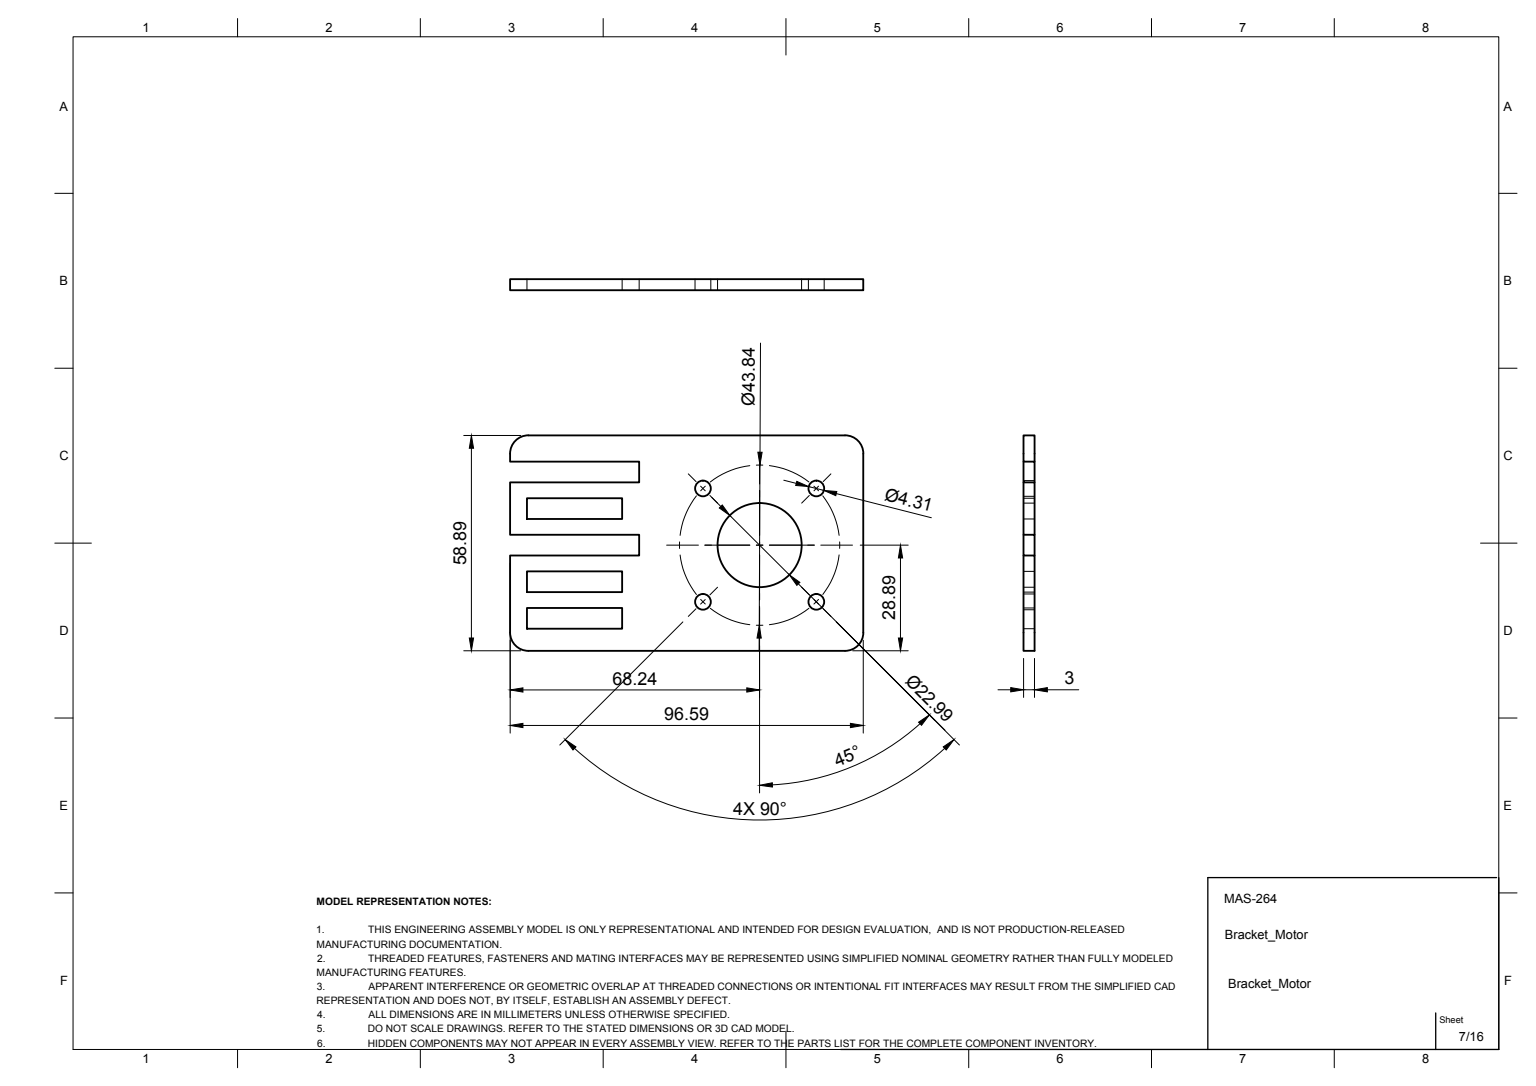
ISO-10303-21;
HEADER;
/* Generated by software containing ST-Developer
 * from STEP Tools, Inc. (www.steptools.com) 
 */

FILE_DESCRIPTION(
/* description */ (''),
/* implementation_level */ '2;1');

FILE_NAME(
/* name */ 'Bracket_Motor.step',
/* time_stamp */ '2026-10-12T15:37:13-07:00',
/* author */ (''),
/* organization */ (''),
/* preprocessor_version */ 'ST-DEVELOPER v20.2',
/* originating_system */ 'Autodesk Translation Framework v15.15.0.0',
/* authorisation */ '');

FILE_SCHEMA (('AUTOMOTIVE_DESIGN { 1 0 10303 214 3 1 1 }'));
ENDSEC;

DATA;
#10=MECHANICAL_DESIGN_GEOMETRIC_PRESENTATION_REPRESENTATION('',(#352),#36460);
#113=SHAPE_REPRESENTATION_RELATIONSHIP('SRR','None',#36525,#126);
#126=ADVANCED_BREP_SHAPE_REPRESENTATION('',(#384),#36454);
#182=FACE_BOUND('',#2191,.T.);
#183=FACE_BOUND('',#2192,.T.);
#184=FACE_BOUND('',#2193,.T.);
#185=FACE_BOUND('',#2194,.T.);
#186=FACE_BOUND('',#2195,.T.);
#187=FACE_BOUND('',#2196,.T.);
#188=FACE_BOUND('',#2197,.T.);
#189=FACE_BOUND('',#2198,.T.);
#190=FACE_BOUND('',#2200,.T.);
#191=FACE_BOUND('',#2201,.T.);
#192=FACE_BOUND('',#2202,.T.);
#193=FACE_BOUND('',#2203,.T.);
#194=FACE_BOUND('',#2204,.T.);
#195=FACE_BOUND('',#2205,.T.);
#196=FACE_BOUND('',#2206,.T.);
#197=FACE_BOUND('',#2207,.T.);
#352=STYLED_ITEM('',(#36596),#384);
#384=MANIFOLD_SOLID_BREP('Body1',#11288);
#634=PLANE('',#12139);
#635=PLANE('',#12140);
#636=PLANE('',#12141);
#637=PLANE('',#12142);
#638=PLANE('',#12143);
#639=PLANE('',#12144);
#640=PLANE('',#12145);
#641=PLANE('',#12146);
#642=PLANE('',#12153);
#643=PLANE('',#12154);
#644=PLANE('',#12155);
#645=PLANE('',#12156);
#646=PLANE('',#12163);
#647=PLANE('',#12164);
#648=PLANE('',#12165);
#649=PLANE('',#12166);
#650=PLANE('',#12167);
#651=PLANE('',#12168);
#652=PLANE('',#12169);
#653=PLANE('',#12170);
#654=PLANE('',#12171);
#655=PLANE('',#12175);
#656=PLANE('',#12179);
#657=PLANE('',#12183);
#658=PLANE('',#12187);
#659=PLANE('',#12188);
#1493=FACE_OUTER_BOUND('',#2157,.T.);
#1494=FACE_OUTER_BOUND('',#2158,.T.);
#1495=FACE_OUTER_BOUND('',#2159,.T.);
#1496=FACE_OUTER_BOUND('',#2160,.T.);
#1497=FACE_OUTER_BOUND('',#2161,.T.);
#1498=FACE_OUTER_BOUND('',#2162,.T.);
#1499=FACE_OUTER_BOUND('',#2163,.T.);
#1500=FACE_OUTER_BOUND('',#2164,.T.);
#1501=FACE_OUTER_BOUND('',#2165,.T.);
#1502=FACE_OUTER_BOUND('',#2166,.T.);
#1503=FACE_OUTER_BOUND('',#2167,.T.);
#1504=FACE_OUTER_BOUND('',#2168,.T.);
#1505=FACE_OUTER_BOUND('',#2169,.T.);
#1506=FACE_OUTER_BOUND('',#2170,.T.);
#1507=FACE_OUTER_BOUND('',#2171,.T.);
#1508=FACE_OUTER_BOUND('',#2172,.T.);
#1509=FACE_OUTER_BOUND('',#2173,.T.);
#1510=FACE_OUTER_BOUND('',#2174,.T.);
#1511=FACE_OUTER_BOUND('',#2175,.T.);
#1512=FACE_OUTER_BOUND('',#2176,.T.);
#1513=FACE_OUTER_BOUND('',#2177,.T.);
#1514=FACE_OUTER_BOUND('',#2178,.T.);
#1515=FACE_OUTER_BOUND('',#2179,.T.);
#1516=FACE_OUTER_BOUND('',#2180,.T.);
#1517=FACE_OUTER_BOUND('',#2181,.T.);
#1518=FACE_OUTER_BOUND('',#2182,.T.);
#1519=FACE_OUTER_BOUND('',#2183,.T.);
#1520=FACE_OUTER_BOUND('',#2184,.T.);
#1521=FACE_OUTER_BOUND('',#2185,.T.);
#1522=FACE_OUTER_BOUND('',#2186,.T.);
#1523=FACE_OUTER_BOUND('',#2187,.T.);
#1524=FACE_OUTER_BOUND('',#2188,.T.);
#1525=FACE_OUTER_BOUND('',#2189,.T.);
#1526=FACE_OUTER_BOUND('',#2190,.T.);
#1527=FACE_OUTER_BOUND('',#2199,.T.);
#2157=EDGE_LOOP('',(#9638,#9639,#9640,#9641));
#2158=EDGE_LOOP('',(#9642,#9643,#9644,#9645));
#2159=EDGE_LOOP('',(#9646,#9647,#9648,#9649));
#2160=EDGE_LOOP('',(#9650,#9651,#9652,#9653));
#2161=EDGE_LOOP('',(#9654,#9655,#9656,#9657));
#2162=EDGE_LOOP('',(#9658,#9659,#9660,#9661));
#2163=EDGE_LOOP('',(#9662,#9663,#9664,#9665));
#2164=EDGE_LOOP('',(#9666,#9667,#9668,#9669));
#2165=EDGE_LOOP('',(#9670,#9671,#9672,#9673));
#2166=EDGE_LOOP('',(#9674,#9675,#9676,#9677));
#2167=EDGE_LOOP('',(#9678,#9679,#9680,#9681));
#2168=EDGE_LOOP('',(#9682,#9683,#9684,#9685));
#2169=EDGE_LOOP('',(#9686,#9687,#9688,#9689));
#2170=EDGE_LOOP('',(#9690,#9691,#9692,#9693));
#2171=EDGE_LOOP('',(#9694,#9695,#9696,#9697));
#2172=EDGE_LOOP('',(#9698,#9699,#9700,#9701));
#2173=EDGE_LOOP('',(#9702,#9703,#9704,#9705));
#2174=EDGE_LOOP('',(#9706,#9707,#9708,#9709));
#2175=EDGE_LOOP('',(#9710,#9711,#9712,#9713));
#2176=EDGE_LOOP('',(#9714,#9715,#9716,#9717));
#2177=EDGE_LOOP('',(#9718,#9719,#9720,#9721));
#2178=EDGE_LOOP('',(#9722,#9723,#9724,#9725));
#2179=EDGE_LOOP('',(#9726,#9727,#9728,#9729));
#2180=EDGE_LOOP('',(#9730,#9731,#9732,#9733));
#2181=EDGE_LOOP('',(#9734,#9735,#9736,#9737));
#2182=EDGE_LOOP('',(#9738,#9739,#9740,#9741));
#2183=EDGE_LOOP('',(#9742,#9743,#9744,#9745));
#2184=EDGE_LOOP('',(#9746,#9747,#9748,#9749));
#2185=EDGE_LOOP('',(#9750,#9751,#9752,#9753));
#2186=EDGE_LOOP('',(#9754,#9755,#9756,#9757));
#2187=EDGE_LOOP('',(#9758,#9759,#9760,#9761));
#2188=EDGE_LOOP('',(#9762,#9763,#9764,#9765));
#2189=EDGE_LOOP('',(#9766,#9767,#9768,#9769));
#2190=EDGE_LOOP('',(#9770,#9771,#9772,#9773,#9774,#9775,#9776,#9777,#9778,
#9779,#9780,#9781,#9782,#9783,#9784,#9785));
#2191=EDGE_LOOP('',(#9786));
#2192=EDGE_LOOP('',(#9787));
#2193=EDGE_LOOP('',(#9788,#9789,#9790,#9791));
#2194=EDGE_LOOP('',(#9792));
#2195=EDGE_LOOP('',(#9793));
#2196=EDGE_LOOP('',(#9794,#9795,#9796,#9797));
#2197=EDGE_LOOP('',(#9798,#9799,#9800,#9801));
#2198=EDGE_LOOP('',(#9802));
#2199=EDGE_LOOP('',(#9803,#9804,#9805,#9806,#9807,#9808,#9809,#9810,#9811,
#9812,#9813,#9814,#9815,#9816,#9817,#9818));
#2200=EDGE_LOOP('',(#9819));
#2201=EDGE_LOOP('',(#9820));
#2202=EDGE_LOOP('',(#9821,#9822,#9823,#9824));
#2203=EDGE_LOOP('',(#9825));
#2204=EDGE_LOOP('',(#9826));
#2205=EDGE_LOOP('',(#9827,#9828,#9829,#9830));
#2206=EDGE_LOOP('',(#9831,#9832,#9833,#9834));
#2207=EDGE_LOOP('',(#9835));
#3086=LINE('',#35485,#4032);
#3087=LINE('',#35490,#4033);
#3088=LINE('',#35492,#4034);
#3089=LINE('',#35494,#4035);
#3090=LINE('',#35495,#4036);
#3091=LINE('',#35498,#4037);
#3092=LINE('',#35500,#4038);
#3093=LINE('',#35501,#4039);
#3094=LINE('',#35504,#4040);
#3095=LINE('',#35506,#4041);
#3096=LINE('',#35507,#4042);
#3097=LINE('',#35509,#4043);
#3098=LINE('',#35510,#4044);
#3099=LINE('',#35514,#4045);
#3100=LINE('',#35516,#4046);
#3101=LINE('',#35518,#4047);
#3102=LINE('',#35519,#4048);
#3103=LINE('',#35522,#4049);
#3104=LINE('',#35524,#4050);
#3105=LINE('',#35525,#4051);
#3106=LINE('',#35528,#4052);
#3107=LINE('',#35530,#4053);
#3108=LINE('',#35531,#4054);
#3109=LINE('',#35533,#4055);
#3110=LINE('',#35534,#4056);
#3111=LINE('',#35539,#4057);
#3112=LINE('',#35545,#4058);
#3113=LINE('',#35550,#4059);
#3114=LINE('',#35552,#4060);
#3115=LINE('',#35554,#4061);
#3116=LINE('',#35555,#4062);
#3117=LINE('',#35558,#4063);
#3118=LINE('',#35560,#4064);
#3119=LINE('',#35561,#4065);
#3120=LINE('',#35564,#4066);
#3121=LINE('',#35566,#4067);
#3122=LINE('',#35567,#4068);
#3123=LINE('',#35569,#4069);
#3124=LINE('',#35570,#4070);
#3125=LINE('',#35575,#4071);
#3126=LINE('',#35581,#4072);
#3127=LINE('',#35586,#4073);
#3128=LINE('',#35588,#4074);
#3129=LINE('',#35590,#4075);
#3130=LINE('',#35591,#4076);
#3131=LINE('',#35594,#4077);
#3132=LINE('',#35596,#4078);
#3133=LINE('',#35597,#4079);
#3134=LINE('',#35600,#4080);
#3135=LINE('',#35602,#4081);
#3136=LINE('',#35603,#4082);
#3137=LINE('',#35606,#4083);
#3138=LINE('',#35608,#4084);
#3139=LINE('',#35609,#4085);
#3140=LINE('',#35612,#4086);
#3141=LINE('',#35614,#4087);
#3142=LINE('',#35615,#4088);
#3143=LINE('',#35618,#4089);
#3144=LINE('',#35620,#4090);
#3145=LINE('',#35621,#4091);
#3146=LINE('',#35624,#4092);
#3147=LINE('',#35626,#4093);
#3148=LINE('',#35627,#4094);
#3149=LINE('',#35630,#4095);
#3150=LINE('',#35632,#4096);
#3151=LINE('',#35633,#4097);
#3152=LINE('',#35636,#4098);
#3153=LINE('',#35638,#4099);
#3154=LINE('',#35639,#4100);
#3155=LINE('',#35645,#4101);
#3156=LINE('',#35648,#4102);
#3157=LINE('',#35650,#4103);
#3158=LINE('',#35651,#4104);
#3159=LINE('',#35657,#4105);
#3160=LINE('',#35660,#4106);
#3161=LINE('',#35662,#4107);
#3162=LINE('',#35663,#4108);
#3163=LINE('',#35669,#4109);
#3164=LINE('',#35672,#4110);
#3165=LINE('',#35674,#4111);
#3166=LINE('',#35675,#4112);
#4032=VECTOR('',#14535,2.155);
#4033=VECTOR('',#14540,10.);
#4034=VECTOR('',#14541,10.);
#4035=VECTOR('',#14542,10.);
#4036=VECTOR('',#14543,10.);
#4037=VECTOR('',#14546,10.);
#4038=VECTOR('',#14547,10.);
#4039=VECTOR('',#14548,10.);
#4040=VECTOR('',#14551,10.);
#4041=VECTOR('',#14552,10.);
#4042=VECTOR('',#14553,10.);
#4043=VECTOR('',#14556,10.);
#4044=VECTOR('',#14557,10.);
#4045=VECTOR('',#14560,10.);
#4046=VECTOR('',#14561,10.);
#4047=VECTOR('',#14562,10.);
#4048=VECTOR('',#14563,10.);
#4049=VECTOR('',#14566,10.);
#4050=VECTOR('',#14567,10.);
#4051=VECTOR('',#14568,10.);
#4052=VECTOR('',#14571,10.);
#4053=VECTOR('',#14572,10.);
#4054=VECTOR('',#14573,10.);
#4055=VECTOR('',#14576,10.);
#4056=VECTOR('',#14577,10.);
#4057=VECTOR('',#14582,2.155);
#4058=VECTOR('',#14589,2.155);
#4059=VECTOR('',#14594,10.);
#4060=VECTOR('',#14595,10.);
#4061=VECTOR('',#14596,10.);
#4062=VECTOR('',#14597,10.);
#4063=VECTOR('',#14600,10.);
#4064=VECTOR('',#14601,10.);
#4065=VECTOR('',#14602,10.);
#4066=VECTOR('',#14605,10.);
#4067=VECTOR('',#14606,10.);
#4068=VECTOR('',#14607,10.);
#4069=VECTOR('',#14610,10.);
#4070=VECTOR('',#14611,10.);
#4071=VECTOR('',#14616,11.493);
#4072=VECTOR('',#14623,2.155);
#4073=VECTOR('',#14628,10.);
#4074=VECTOR('',#14629,10.);
#4075=VECTOR('',#14630,10.);
#4076=VECTOR('',#14631,10.);
#4077=VECTOR('',#14634,10.);
#4078=VECTOR('',#14635,10.);
#4079=VECTOR('',#14636,10.);
#4080=VECTOR('',#14639,10.);
#4081=VECTOR('',#14640,10.);
#4082=VECTOR('',#14641,10.);
#4083=VECTOR('',#14644,10.);
#4084=VECTOR('',#14645,10.);
#4085=VECTOR('',#14646,10.);
#4086=VECTOR('',#14649,10.);
#4087=VECTOR('',#14650,10.);
#4088=VECTOR('',#14651,10.);
#4089=VECTOR('',#14654,10.);
#4090=VECTOR('',#14655,10.);
#4091=VECTOR('',#14656,10.);
#4092=VECTOR('',#14659,10.);
#4093=VECTOR('',#14660,10.);
#4094=VECTOR('',#14661,10.);
#4095=VECTOR('',#14664,10.);
#4096=VECTOR('',#14665,10.);
#4097=VECTOR('',#14666,10.);
#4098=VECTOR('',#14669,10.);
#4099=VECTOR('',#14670,10.);
#4100=VECTOR('',#14671,10.);
#4101=VECTOR('',#14678,10.);
#4102=VECTOR('',#14681,10.);
#4103=VECTOR('',#14682,10.);
#4104=VECTOR('',#14683,10.);
#4105=VECTOR('',#14690,10.);
#4106=VECTOR('',#14693,10.);
#4107=VECTOR('',#14694,10.);
#4108=VECTOR('',#14695,10.);
#4109=VECTOR('',#14702,10.);
#4110=VECTOR('',#14705,10.);
#4111=VECTOR('',#14706,10.);
#4112=VECTOR('',#14707,10.);
#4461=CIRCLE('',#12137,2.155);
#4462=CIRCLE('',#12138,2.155);
#4463=CIRCLE('',#12148,2.155);
#4464=CIRCLE('',#12149,2.155);
#4465=CIRCLE('',#12151,2.155);
#4466=CIRCLE('',#12152,2.155);
#4467=CIRCLE('',#12158,11.493);
#4468=CIRCLE('',#12159,11.493);
#4469=CIRCLE('',#12161,2.155);
#4470=CIRCLE('',#12162,2.155);
#4471=CIRCLE('',#12173,5.);
#4472=CIRCLE('',#12174,5.);
#4473=CIRCLE('',#12177,5.00000000000002);
#4474=CIRCLE('',#12178,5.00000000000002);
#4475=CIRCLE('',#12181,5.);
#4476=CIRCLE('',#12182,5.);
#4477=CIRCLE('',#12185,4.99999999999999);
#4478=CIRCLE('',#12186,4.99999999999999);
#5395=VERTEX_POINT('',#35482);
#5396=VERTEX_POINT('',#35484);
#5397=VERTEX_POINT('',#35488);
#5398=VERTEX_POINT('',#35489);
#5399=VERTEX_POINT('',#35491);
#5400=VERTEX_POINT('',#35493);
#5401=VERTEX_POINT('',#35497);
#5402=VERTEX_POINT('',#35499);
#5403=VERTEX_POINT('',#35503);
#5404=VERTEX_POINT('',#35505);
#5405=VERTEX_POINT('',#35512);
#5406=VERTEX_POINT('',#35513);
#5407=VERTEX_POINT('',#35515);
#5408=VERTEX_POINT('',#35517);
#5409=VERTEX_POINT('',#35521);
#5410=VERTEX_POINT('',#35523);
#5411=VERTEX_POINT('',#35527);
#5412=VERTEX_POINT('',#35529);
#5413=VERTEX_POINT('',#35536);
#5414=VERTEX_POINT('',#35538);
#5415=VERTEX_POINT('',#35542);
#5416=VERTEX_POINT('',#35544);
#5417=VERTEX_POINT('',#35548);
#5418=VERTEX_POINT('',#35549);
#5419=VERTEX_POINT('',#35551);
#5420=VERTEX_POINT('',#35553);
#5421=VERTEX_POINT('',#35557);
#5422=VERTEX_POINT('',#35559);
#5423=VERTEX_POINT('',#35563);
#5424=VERTEX_POINT('',#35565);
#5425=VERTEX_POINT('',#35572);
#5426=VERTEX_POINT('',#35574);
#5427=VERTEX_POINT('',#35578);
#5428=VERTEX_POINT('',#35580);
#5429=VERTEX_POINT('',#35584);
#5430=VERTEX_POINT('',#35585);
#5431=VERTEX_POINT('',#35587);
#5432=VERTEX_POINT('',#35589);
#5433=VERTEX_POINT('',#35593);
#5434=VERTEX_POINT('',#35595);
#5435=VERTEX_POINT('',#35599);
#5436=VERTEX_POINT('',#35601);
#5437=VERTEX_POINT('',#35605);
#5438=VERTEX_POINT('',#35607);
#5439=VERTEX_POINT('',#35611);
#5440=VERTEX_POINT('',#35613);
#5441=VERTEX_POINT('',#35617);
#5442=VERTEX_POINT('',#35619);
#5443=VERTEX_POINT('',#35623);
#5444=VERTEX_POINT('',#35625);
#5445=VERTEX_POINT('',#35629);
#5446=VERTEX_POINT('',#35631);
#5447=VERTEX_POINT('',#35635);
#5448=VERTEX_POINT('',#35637);
#5449=VERTEX_POINT('',#35641);
#5450=VERTEX_POINT('',#35643);
#5451=VERTEX_POINT('',#35647);
#5452=VERTEX_POINT('',#35649);
#5453=VERTEX_POINT('',#35653);
#5454=VERTEX_POINT('',#35655);
#5455=VERTEX_POINT('',#35659);
#5456=VERTEX_POINT('',#35661);
#5457=VERTEX_POINT('',#35665);
#5458=VERTEX_POINT('',#35667);
#5459=VERTEX_POINT('',#35671);
#5460=VERTEX_POINT('',#35673);
#6850=EDGE_CURVE('',#5395,#5395,#4461,.T.);
#6851=EDGE_CURVE('',#5395,#5396,#3086,.T.);
#6852=EDGE_CURVE('',#5396,#5396,#4462,.T.);
#6853=EDGE_CURVE('',#5397,#5398,#3087,.T.);
#6854=EDGE_CURVE('',#5398,#5399,#3088,.T.);
#6855=EDGE_CURVE('',#5400,#5399,#3089,.T.);
#6856=EDGE_CURVE('',#5397,#5400,#3090,.T.);
#6857=EDGE_CURVE('',#5401,#5397,#3091,.T.);
#6858=EDGE_CURVE('',#5402,#5400,#3092,.T.);
#6859=EDGE_CURVE('',#5401,#5402,#3093,.T.);
#6860=EDGE_CURVE('',#5403,#5401,#3094,.T.);
#6861=EDGE_CURVE('',#5404,#5402,#3095,.T.);
#6862=EDGE_CURVE('',#5403,#5404,#3096,.T.);
#6863=EDGE_CURVE('',#5398,#5403,#3097,.T.);
#6864=EDGE_CURVE('',#5399,#5404,#3098,.T.);
#6865=EDGE_CURVE('',#5405,#5406,#3099,.T.);
#6866=EDGE_CURVE('',#5406,#5407,#3100,.T.);
#6867=EDGE_CURVE('',#5408,#5407,#3101,.T.);
#6868=EDGE_CURVE('',#5405,#5408,#3102,.T.);
#6869=EDGE_CURVE('',#5409,#5405,#3103,.T.);
#6870=EDGE_CURVE('',#5410,#5408,#3104,.T.);
#6871=EDGE_CURVE('',#5409,#5410,#3105,.T.);
#6872=EDGE_CURVE('',#5411,#5409,#3106,.T.);
#6873=EDGE_CURVE('',#5412,#5410,#3107,.T.);
#6874=EDGE_CURVE('',#5411,#5412,#3108,.T.);
#6875=EDGE_CURVE('',#5406,#5411,#3109,.T.);
#6876=EDGE_CURVE('',#5407,#5412,#3110,.T.);
#6877=EDGE_CURVE('',#5413,#5413,#4463,.T.);
#6878=EDGE_CURVE('',#5413,#5414,#3111,.T.);
#6879=EDGE_CURVE('',#5414,#5414,#4464,.T.);
#6880=EDGE_CURVE('',#5415,#5415,#4465,.T.);
#6881=EDGE_CURVE('',#5415,#5416,#3112,.T.);
#6882=EDGE_CURVE('',#5416,#5416,#4466,.T.);
#6883=EDGE_CURVE('',#5417,#5418,#3113,.T.);
#6884=EDGE_CURVE('',#5418,#5419,#3114,.T.);
#6885=EDGE_CURVE('',#5420,#5419,#3115,.T.);
#6886=EDGE_CURVE('',#5417,#5420,#3116,.T.);
#6887=EDGE_CURVE('',#5421,#5417,#3117,.T.);
#6888=EDGE_CURVE('',#5422,#5420,#3118,.T.);
#6889=EDGE_CURVE('',#5421,#5422,#3119,.T.);
#6890=EDGE_CURVE('',#5423,#5421,#3120,.T.);
#6891=EDGE_CURVE('',#5424,#5422,#3121,.T.);
#6892=EDGE_CURVE('',#5423,#5424,#3122,.T.);
#6893=EDGE_CURVE('',#5418,#5423,#3123,.T.);
#6894=EDGE_CURVE('',#5419,#5424,#3124,.T.);
#6895=EDGE_CURVE('',#5425,#5425,#4467,.T.);
#6896=EDGE_CURVE('',#5425,#5426,#3125,.T.);
#6897=EDGE_CURVE('',#5426,#5426,#4468,.T.);
#6898=EDGE_CURVE('',#5427,#5427,#4469,.T.);
#6899=EDGE_CURVE('',#5427,#5428,#3126,.T.);
#6900=EDGE_CURVE('',#5428,#5428,#4470,.T.);
#6901=EDGE_CURVE('',#5429,#5430,#3127,.T.);
#6902=EDGE_CURVE('',#5429,#5431,#3128,.T.);
#6903=EDGE_CURVE('',#5432,#5431,#3129,.T.);
#6904=EDGE_CURVE('',#5430,#5432,#3130,.T.);
#6905=EDGE_CURVE('',#5430,#5433,#3131,.T.);
#6906=EDGE_CURVE('',#5434,#5432,#3132,.T.);
#6907=EDGE_CURVE('',#5433,#5434,#3133,.T.);
#6908=EDGE_CURVE('',#5433,#5435,#3134,.T.);
#6909=EDGE_CURVE('',#5436,#5434,#3135,.T.);
#6910=EDGE_CURVE('',#5435,#5436,#3136,.T.);
#6911=EDGE_CURVE('',#5435,#5437,#3137,.T.);
#6912=EDGE_CURVE('',#5438,#5436,#3138,.T.);
#6913=EDGE_CURVE('',#5437,#5438,#3139,.T.);
#6914=EDGE_CURVE('',#5437,#5439,#3140,.T.);
#6915=EDGE_CURVE('',#5440,#5438,#3141,.T.);
#6916=EDGE_CURVE('',#5439,#5440,#3142,.T.);
#6917=EDGE_CURVE('',#5439,#5441,#3143,.T.);
#6918=EDGE_CURVE('',#5442,#5440,#3144,.T.);
#6919=EDGE_CURVE('',#5441,#5442,#3145,.T.);
#6920=EDGE_CURVE('',#5441,#5443,#3146,.T.);
#6921=EDGE_CURVE('',#5444,#5442,#3147,.T.);
#6922=EDGE_CURVE('',#5443,#5444,#3148,.T.);
#6923=EDGE_CURVE('',#5443,#5445,#3149,.T.);
#6924=EDGE_CURVE('',#5446,#5444,#3150,.T.);
#6925=EDGE_CURVE('',#5445,#5446,#3151,.T.);
#6926=EDGE_CURVE('',#5445,#5447,#3152,.T.);
#6927=EDGE_CURVE('',#5448,#5446,#3153,.T.);
#6928=EDGE_CURVE('',#5447,#5448,#3154,.T.);
#6929=EDGE_CURVE('',#5449,#5447,#4471,.T.);
#6930=EDGE_CURVE('',#5450,#5448,#4472,.T.);
#6931=EDGE_CURVE('',#5449,#5450,#3155,.T.);
#6932=EDGE_CURVE('',#5449,#5451,#3156,.T.);
#6933=EDGE_CURVE('',#5452,#5450,#3157,.T.);
#6934=EDGE_CURVE('',#5451,#5452,#3158,.T.);
#6935=EDGE_CURVE('',#5453,#5451,#4473,.T.);
#6936=EDGE_CURVE('',#5454,#5452,#4474,.T.);
#6937=EDGE_CURVE('',#5453,#5454,#3159,.T.);
#6938=EDGE_CURVE('',#5453,#5455,#3160,.T.);
#6939=EDGE_CURVE('',#5456,#5454,#3161,.T.);
#6940=EDGE_CURVE('',#5455,#5456,#3162,.T.);
#6941=EDGE_CURVE('',#5457,#5455,#4475,.T.);
#6942=EDGE_CURVE('',#5458,#5456,#4476,.T.);
#6943=EDGE_CURVE('',#5457,#5458,#3163,.T.);
#6944=EDGE_CURVE('',#5457,#5459,#3164,.T.);
#6945=EDGE_CURVE('',#5460,#5458,#3165,.T.);
#6946=EDGE_CURVE('',#5459,#5460,#3166,.T.);
#6947=EDGE_CURVE('',#5429,#5459,#4477,.T.);
#6948=EDGE_CURVE('',#5431,#5460,#4478,.T.);
#9638=ORIENTED_EDGE('',*,*,#6850,.T.);
#9639=ORIENTED_EDGE('',*,*,#6851,.T.);
#9640=ORIENTED_EDGE('',*,*,#6852,.F.);
#9641=ORIENTED_EDGE('',*,*,#6851,.F.);
#9642=ORIENTED_EDGE('',*,*,#6853,.T.);
#9643=ORIENTED_EDGE('',*,*,#6854,.T.);
#9644=ORIENTED_EDGE('',*,*,#6855,.F.);
#9645=ORIENTED_EDGE('',*,*,#6856,.F.);
#9646=ORIENTED_EDGE('',*,*,#6857,.T.);
#9647=ORIENTED_EDGE('',*,*,#6856,.T.);
#9648=ORIENTED_EDGE('',*,*,#6858,.F.);
#9649=ORIENTED_EDGE('',*,*,#6859,.F.);
#9650=ORIENTED_EDGE('',*,*,#6860,.T.);
#9651=ORIENTED_EDGE('',*,*,#6859,.T.);
#9652=ORIENTED_EDGE('',*,*,#6861,.F.);
#9653=ORIENTED_EDGE('',*,*,#6862,.F.);
#9654=ORIENTED_EDGE('',*,*,#6863,.T.);
#9655=ORIENTED_EDGE('',*,*,#6862,.T.);
#9656=ORIENTED_EDGE('',*,*,#6864,.F.);
#9657=ORIENTED_EDGE('',*,*,#6854,.F.);
#9658=ORIENTED_EDGE('',*,*,#6865,.T.);
#9659=ORIENTED_EDGE('',*,*,#6866,.T.);
#9660=ORIENTED_EDGE('',*,*,#6867,.F.);
#9661=ORIENTED_EDGE('',*,*,#6868,.F.);
#9662=ORIENTED_EDGE('',*,*,#6869,.T.);
#9663=ORIENTED_EDGE('',*,*,#6868,.T.);
#9664=ORIENTED_EDGE('',*,*,#6870,.F.);
#9665=ORIENTED_EDGE('',*,*,#6871,.F.);
#9666=ORIENTED_EDGE('',*,*,#6872,.T.);
#9667=ORIENTED_EDGE('',*,*,#6871,.T.);
#9668=ORIENTED_EDGE('',*,*,#6873,.F.);
#9669=ORIENTED_EDGE('',*,*,#6874,.F.);
#9670=ORIENTED_EDGE('',*,*,#6875,.T.);
#9671=ORIENTED_EDGE('',*,*,#6874,.T.);
#9672=ORIENTED_EDGE('',*,*,#6876,.F.);
#9673=ORIENTED_EDGE('',*,*,#6866,.F.);
#9674=ORIENTED_EDGE('',*,*,#6877,.T.);
#9675=ORIENTED_EDGE('',*,*,#6878,.T.);
#9676=ORIENTED_EDGE('',*,*,#6879,.F.);
#9677=ORIENTED_EDGE('',*,*,#6878,.F.);
#9678=ORIENTED_EDGE('',*,*,#6880,.T.);
#9679=ORIENTED_EDGE('',*,*,#6881,.T.);
#9680=ORIENTED_EDGE('',*,*,#6882,.F.);
#9681=ORIENTED_EDGE('',*,*,#6881,.F.);
#9682=ORIENTED_EDGE('',*,*,#6883,.T.);
#9683=ORIENTED_EDGE('',*,*,#6884,.T.);
#9684=ORIENTED_EDGE('',*,*,#6885,.F.);
#9685=ORIENTED_EDGE('',*,*,#6886,.F.);
#9686=ORIENTED_EDGE('',*,*,#6887,.T.);
#9687=ORIENTED_EDGE('',*,*,#6886,.T.);
#9688=ORIENTED_EDGE('',*,*,#6888,.F.);
#9689=ORIENTED_EDGE('',*,*,#6889,.F.);
#9690=ORIENTED_EDGE('',*,*,#6890,.T.);
#9691=ORIENTED_EDGE('',*,*,#6889,.T.);
#9692=ORIENTED_EDGE('',*,*,#6891,.F.);
#9693=ORIENTED_EDGE('',*,*,#6892,.F.);
#9694=ORIENTED_EDGE('',*,*,#6893,.T.);
#9695=ORIENTED_EDGE('',*,*,#6892,.T.);
#9696=ORIENTED_EDGE('',*,*,#6894,.F.);
#9697=ORIENTED_EDGE('',*,*,#6884,.F.);
#9698=ORIENTED_EDGE('',*,*,#6895,.T.);
#9699=ORIENTED_EDGE('',*,*,#6896,.T.);
#9700=ORIENTED_EDGE('',*,*,#6897,.F.);
#9701=ORIENTED_EDGE('',*,*,#6896,.F.);
#9702=ORIENTED_EDGE('',*,*,#6898,.T.);
#9703=ORIENTED_EDGE('',*,*,#6899,.T.);
#9704=ORIENTED_EDGE('',*,*,#6900,.F.);
#9705=ORIENTED_EDGE('',*,*,#6899,.F.);
#9706=ORIENTED_EDGE('',*,*,#6901,.F.);
#9707=ORIENTED_EDGE('',*,*,#6902,.T.);
#9708=ORIENTED_EDGE('',*,*,#6903,.F.);
#9709=ORIENTED_EDGE('',*,*,#6904,.F.);
#9710=ORIENTED_EDGE('',*,*,#6905,.F.);
#9711=ORIENTED_EDGE('',*,*,#6904,.T.);
#9712=ORIENTED_EDGE('',*,*,#6906,.F.);
#9713=ORIENTED_EDGE('',*,*,#6907,.F.);
#9714=ORIENTED_EDGE('',*,*,#6908,.F.);
#9715=ORIENTED_EDGE('',*,*,#6907,.T.);
#9716=ORIENTED_EDGE('',*,*,#6909,.F.);
#9717=ORIENTED_EDGE('',*,*,#6910,.F.);
#9718=ORIENTED_EDGE('',*,*,#6911,.F.);
#9719=ORIENTED_EDGE('',*,*,#6910,.T.);
#9720=ORIENTED_EDGE('',*,*,#6912,.F.);
#9721=ORIENTED_EDGE('',*,*,#6913,.F.);
#9722=ORIENTED_EDGE('',*,*,#6914,.F.);
#9723=ORIENTED_EDGE('',*,*,#6913,.T.);
#9724=ORIENTED_EDGE('',*,*,#6915,.F.);
#9725=ORIENTED_EDGE('',*,*,#6916,.F.);
#9726=ORIENTED_EDGE('',*,*,#6917,.F.);
#9727=ORIENTED_EDGE('',*,*,#6916,.T.);
#9728=ORIENTED_EDGE('',*,*,#6918,.F.);
#9729=ORIENTED_EDGE('',*,*,#6919,.F.);
#9730=ORIENTED_EDGE('',*,*,#6920,.F.);
#9731=ORIENTED_EDGE('',*,*,#6919,.T.);
#9732=ORIENTED_EDGE('',*,*,#6921,.F.);
#9733=ORIENTED_EDGE('',*,*,#6922,.F.);
#9734=ORIENTED_EDGE('',*,*,#6923,.F.);
#9735=ORIENTED_EDGE('',*,*,#6922,.T.);
#9736=ORIENTED_EDGE('',*,*,#6924,.F.);
#9737=ORIENTED_EDGE('',*,*,#6925,.F.);
#9738=ORIENTED_EDGE('',*,*,#6926,.F.);
#9739=ORIENTED_EDGE('',*,*,#6925,.T.);
#9740=ORIENTED_EDGE('',*,*,#6927,.F.);
#9741=ORIENTED_EDGE('',*,*,#6928,.F.);
#9742=ORIENTED_EDGE('',*,*,#6929,.T.);
#9743=ORIENTED_EDGE('',*,*,#6928,.T.);
#9744=ORIENTED_EDGE('',*,*,#6930,.F.);
#9745=ORIENTED_EDGE('',*,*,#6931,.F.);
#9746=ORIENTED_EDGE('',*,*,#6932,.F.);
#9747=ORIENTED_EDGE('',*,*,#6931,.T.);
#9748=ORIENTED_EDGE('',*,*,#6933,.F.);
#9749=ORIENTED_EDGE('',*,*,#6934,.F.);
#9750=ORIENTED_EDGE('',*,*,#6935,.T.);
#9751=ORIENTED_EDGE('',*,*,#6934,.T.);
#9752=ORIENTED_EDGE('',*,*,#6936,.F.);
#9753=ORIENTED_EDGE('',*,*,#6937,.F.);
#9754=ORIENTED_EDGE('',*,*,#6938,.F.);
#9755=ORIENTED_EDGE('',*,*,#6937,.T.);
#9756=ORIENTED_EDGE('',*,*,#6939,.F.);
#9757=ORIENTED_EDGE('',*,*,#6940,.F.);
#9758=ORIENTED_EDGE('',*,*,#6941,.T.);
#9759=ORIENTED_EDGE('',*,*,#6940,.T.);
#9760=ORIENTED_EDGE('',*,*,#6942,.F.);
#9761=ORIENTED_EDGE('',*,*,#6943,.F.);
#9762=ORIENTED_EDGE('',*,*,#6944,.F.);
#9763=ORIENTED_EDGE('',*,*,#6943,.T.);
#9764=ORIENTED_EDGE('',*,*,#6945,.F.);
#9765=ORIENTED_EDGE('',*,*,#6946,.F.);
#9766=ORIENTED_EDGE('',*,*,#6947,.T.);
#9767=ORIENTED_EDGE('',*,*,#6946,.T.);
#9768=ORIENTED_EDGE('',*,*,#6948,.F.);
#9769=ORIENTED_EDGE('',*,*,#6902,.F.);
#9770=ORIENTED_EDGE('',*,*,#6948,.T.);
#9771=ORIENTED_EDGE('',*,*,#6945,.T.);
#9772=ORIENTED_EDGE('',*,*,#6942,.T.);
#9773=ORIENTED_EDGE('',*,*,#6939,.T.);
#9774=ORIENTED_EDGE('',*,*,#6936,.T.);
#9775=ORIENTED_EDGE('',*,*,#6933,.T.);
#9776=ORIENTED_EDGE('',*,*,#6930,.T.);
#9777=ORIENTED_EDGE('',*,*,#6927,.T.);
#9778=ORIENTED_EDGE('',*,*,#6924,.T.);
#9779=ORIENTED_EDGE('',*,*,#6921,.T.);
#9780=ORIENTED_EDGE('',*,*,#6918,.T.);
#9781=ORIENTED_EDGE('',*,*,#6915,.T.);
#9782=ORIENTED_EDGE('',*,*,#6912,.T.);
#9783=ORIENTED_EDGE('',*,*,#6909,.T.);
#9784=ORIENTED_EDGE('',*,*,#6906,.T.);
#9785=ORIENTED_EDGE('',*,*,#6903,.T.);
#9786=ORIENTED_EDGE('',*,*,#6900,.T.);
#9787=ORIENTED_EDGE('',*,*,#6897,.T.);
#9788=ORIENTED_EDGE('',*,*,#6894,.T.);
#9789=ORIENTED_EDGE('',*,*,#6891,.T.);
#9790=ORIENTED_EDGE('',*,*,#6888,.T.);
#9791=ORIENTED_EDGE('',*,*,#6885,.T.);
#9792=ORIENTED_EDGE('',*,*,#6882,.T.);
#9793=ORIENTED_EDGE('',*,*,#6879,.T.);
#9794=ORIENTED_EDGE('',*,*,#6876,.T.);
#9795=ORIENTED_EDGE('',*,*,#6873,.T.);
#9796=ORIENTED_EDGE('',*,*,#6870,.T.);
#9797=ORIENTED_EDGE('',*,*,#6867,.T.);
#9798=ORIENTED_EDGE('',*,*,#6864,.T.);
#9799=ORIENTED_EDGE('',*,*,#6861,.T.);
#9800=ORIENTED_EDGE('',*,*,#6858,.T.);
#9801=ORIENTED_EDGE('',*,*,#6855,.T.);
#9802=ORIENTED_EDGE('',*,*,#6852,.T.);
#9803=ORIENTED_EDGE('',*,*,#6947,.F.);
#9804=ORIENTED_EDGE('',*,*,#6901,.T.);
#9805=ORIENTED_EDGE('',*,*,#6905,.T.);
#9806=ORIENTED_EDGE('',*,*,#6908,.T.);
#9807=ORIENTED_EDGE('',*,*,#6911,.T.);
#9808=ORIENTED_EDGE('',*,*,#6914,.T.);
#9809=ORIENTED_EDGE('',*,*,#6917,.T.);
#9810=ORIENTED_EDGE('',*,*,#6920,.T.);
#9811=ORIENTED_EDGE('',*,*,#6923,.T.);
#9812=ORIENTED_EDGE('',*,*,#6926,.T.);
#9813=ORIENTED_EDGE('',*,*,#6929,.F.);
#9814=ORIENTED_EDGE('',*,*,#6932,.T.);
#9815=ORIENTED_EDGE('',*,*,#6935,.F.);
#9816=ORIENTED_EDGE('',*,*,#6938,.T.);
#9817=ORIENTED_EDGE('',*,*,#6941,.F.);
#9818=ORIENTED_EDGE('',*,*,#6944,.T.);
#9819=ORIENTED_EDGE('',*,*,#6898,.F.);
#9820=ORIENTED_EDGE('',*,*,#6895,.F.);
#9821=ORIENTED_EDGE('',*,*,#6893,.F.);
#9822=ORIENTED_EDGE('',*,*,#6883,.F.);
#9823=ORIENTED_EDGE('',*,*,#6887,.F.);
#9824=ORIENTED_EDGE('',*,*,#6890,.F.);
#9825=ORIENTED_EDGE('',*,*,#6880,.F.);
#9826=ORIENTED_EDGE('',*,*,#6877,.F.);
#9827=ORIENTED_EDGE('',*,*,#6875,.F.);
#9828=ORIENTED_EDGE('',*,*,#6865,.F.);
#9829=ORIENTED_EDGE('',*,*,#6869,.F.);
#9830=ORIENTED_EDGE('',*,*,#6872,.F.);
#9831=ORIENTED_EDGE('',*,*,#6863,.F.);
#9832=ORIENTED_EDGE('',*,*,#6853,.F.);
#9833=ORIENTED_EDGE('',*,*,#6857,.F.);
#9834=ORIENTED_EDGE('',*,*,#6860,.F.);
#9835=ORIENTED_EDGE('',*,*,#6850,.F.);
#10583=CYLINDRICAL_SURFACE('',#12136,2.155);
#10584=CYLINDRICAL_SURFACE('',#12147,2.155);
#10585=CYLINDRICAL_SURFACE('',#12150,2.155);
#10586=CYLINDRICAL_SURFACE('',#12157,11.493);
#10587=CYLINDRICAL_SURFACE('',#12160,2.155);
#10588=CYLINDRICAL_SURFACE('',#12172,5.);
#10589=CYLINDRICAL_SURFACE('',#12176,5.00000000000002);
#10590=CYLINDRICAL_SURFACE('',#12180,5.);
#10591=CYLINDRICAL_SURFACE('',#12184,4.99999999999999);
#11114=ADVANCED_FACE('',(#1493),#10583,.F.);
#11115=ADVANCED_FACE('',(#1494),#634,.T.);
#11116=ADVANCED_FACE('',(#1495),#635,.T.);
#11117=ADVANCED_FACE('',(#1496),#636,.T.);
#11118=ADVANCED_FACE('',(#1497),#637,.T.);
#11119=ADVANCED_FACE('',(#1498),#638,.T.);
#11120=ADVANCED_FACE('',(#1499),#639,.T.);
#11121=ADVANCED_FACE('',(#1500),#640,.T.);
#11122=ADVANCED_FACE('',(#1501),#641,.T.);
#11123=ADVANCED_FACE('',(#1502),#10584,.F.);
#11124=ADVANCED_FACE('',(#1503),#10585,.F.);
#11125=ADVANCED_FACE('',(#1504),#642,.T.);
#11126=ADVANCED_FACE('',(#1505),#643,.T.);
#11127=ADVANCED_FACE('',(#1506),#644,.T.);
#11128=ADVANCED_FACE('',(#1507),#645,.T.);
#11129=ADVANCED_FACE('',(#1508),#10586,.F.);
#11130=ADVANCED_FACE('',(#1509),#10587,.F.);
#11131=ADVANCED_FACE('',(#1510),#646,.T.);
#11132=ADVANCED_FACE('',(#1511),#647,.T.);
#11133=ADVANCED_FACE('',(#1512),#648,.T.);
#11134=ADVANCED_FACE('',(#1513),#649,.T.);
#11135=ADVANCED_FACE('',(#1514),#650,.T.);
#11136=ADVANCED_FACE('',(#1515),#651,.T.);
#11137=ADVANCED_FACE('',(#1516),#652,.T.);
#11138=ADVANCED_FACE('',(#1517),#653,.T.);
#11139=ADVANCED_FACE('',(#1518),#654,.T.);
#11140=ADVANCED_FACE('',(#1519),#10588,.T.);
#11141=ADVANCED_FACE('',(#1520),#655,.T.);
#11142=ADVANCED_FACE('',(#1521),#10589,.T.);
#11143=ADVANCED_FACE('',(#1522),#656,.T.);
#11144=ADVANCED_FACE('',(#1523),#10590,.T.);
#11145=ADVANCED_FACE('',(#1524),#657,.T.);
#11146=ADVANCED_FACE('',(#1525),#10591,.T.);
#11147=ADVANCED_FACE('',(#1526,#182,#183,#184,#185,#186,#187,#188,#189),
#658,.T.);
#11148=ADVANCED_FACE('',(#1527,#190,#191,#192,#193,#194,#195,#196,#197),
#659,.F.);
#11288=CLOSED_SHELL('',(#11114,#11115,#11116,#11117,#11118,#11119,#11120,
#11121,#11122,#11123,#11124,#11125,#11126,#11127,#11128,#11129,#11130,#11131,
#11132,#11133,#11134,#11135,#11136,#11137,#11138,#11139,#11140,#11141,#11142,
#11143,#11144,#11145,#11146,#11147,#11148));
#12135=AXIS2_PLACEMENT_3D('',#35480,#14529,#14530);
#12136=AXIS2_PLACEMENT_3D('',#35481,#14531,#14532);
#12137=AXIS2_PLACEMENT_3D('',#35483,#14533,#14534);
#12138=AXIS2_PLACEMENT_3D('',#35486,#14536,#14537);
#12139=AXIS2_PLACEMENT_3D('',#35487,#14538,#14539);
#12140=AXIS2_PLACEMENT_3D('',#35496,#14544,#14545);
#12141=AXIS2_PLACEMENT_3D('',#35502,#14549,#14550);
#12142=AXIS2_PLACEMENT_3D('',#35508,#14554,#14555);
#12143=AXIS2_PLACEMENT_3D('',#35511,#14558,#14559);
#12144=AXIS2_PLACEMENT_3D('',#35520,#14564,#14565);
#12145=AXIS2_PLACEMENT_3D('',#35526,#14569,#14570);
#12146=AXIS2_PLACEMENT_3D('',#35532,#14574,#14575);
#12147=AXIS2_PLACEMENT_3D('',#35535,#14578,#14579);
#12148=AXIS2_PLACEMENT_3D('',#35537,#14580,#14581);
#12149=AXIS2_PLACEMENT_3D('',#35540,#14583,#14584);
#12150=AXIS2_PLACEMENT_3D('',#35541,#14585,#14586);
#12151=AXIS2_PLACEMENT_3D('',#35543,#14587,#14588);
#12152=AXIS2_PLACEMENT_3D('',#35546,#14590,#14591);
#12153=AXIS2_PLACEMENT_3D('',#35547,#14592,#14593);
#12154=AXIS2_PLACEMENT_3D('',#35556,#14598,#14599);
#12155=AXIS2_PLACEMENT_3D('',#35562,#14603,#14604);
#12156=AXIS2_PLACEMENT_3D('',#35568,#14608,#14609);
#12157=AXIS2_PLACEMENT_3D('',#35571,#14612,#14613);
#12158=AXIS2_PLACEMENT_3D('',#35573,#14614,#14615);
#12159=AXIS2_PLACEMENT_3D('',#35576,#14617,#14618);
#12160=AXIS2_PLACEMENT_3D('',#35577,#14619,#14620);
#12161=AXIS2_PLACEMENT_3D('',#35579,#14621,#14622);
#12162=AXIS2_PLACEMENT_3D('',#35582,#14624,#14625);
#12163=AXIS2_PLACEMENT_3D('',#35583,#14626,#14627);
#12164=AXIS2_PLACEMENT_3D('',#35592,#14632,#14633);
#12165=AXIS2_PLACEMENT_3D('',#35598,#14637,#14638);
#12166=AXIS2_PLACEMENT_3D('',#35604,#14642,#14643);
#12167=AXIS2_PLACEMENT_3D('',#35610,#14647,#14648);
#12168=AXIS2_PLACEMENT_3D('',#35616,#14652,#14653);
#12169=AXIS2_PLACEMENT_3D('',#35622,#14657,#14658);
#12170=AXIS2_PLACEMENT_3D('',#35628,#14662,#14663);
#12171=AXIS2_PLACEMENT_3D('',#35634,#14667,#14668);
#12172=AXIS2_PLACEMENT_3D('',#35640,#14672,#14673);
#12173=AXIS2_PLACEMENT_3D('',#35642,#14674,#14675);
#12174=AXIS2_PLACEMENT_3D('',#35644,#14676,#14677);
#12175=AXIS2_PLACEMENT_3D('',#35646,#14679,#14680);
#12176=AXIS2_PLACEMENT_3D('',#35652,#14684,#14685);
#12177=AXIS2_PLACEMENT_3D('',#35654,#14686,#14687);
#12178=AXIS2_PLACEMENT_3D('',#35656,#14688,#14689);
#12179=AXIS2_PLACEMENT_3D('',#35658,#14691,#14692);
#12180=AXIS2_PLACEMENT_3D('',#35664,#14696,#14697);
#12181=AXIS2_PLACEMENT_3D('',#35666,#14698,#14699);
#12182=AXIS2_PLACEMENT_3D('',#35668,#14700,#14701);
#12183=AXIS2_PLACEMENT_3D('',#35670,#14703,#14704);
#12184=AXIS2_PLACEMENT_3D('',#35676,#14708,#14709);
#12185=AXIS2_PLACEMENT_3D('',#35677,#14710,#14711);
#12186=AXIS2_PLACEMENT_3D('',#35678,#14712,#14713);
#12187=AXIS2_PLACEMENT_3D('',#35679,#14714,#14715);
#12188=AXIS2_PLACEMENT_3D('',#35680,#14716,#14717);
#14529=DIRECTION('axis',(0.,0.,1.));
#14530=DIRECTION('refdir',(1.,0.,0.));
#14531=DIRECTION('center_axis',(7.40148683083437E-16,0.,-1.));
#14532=DIRECTION('ref_axis',(-1.,0.,-7.40148683083437E-16));
#14533=DIRECTION('center_axis',(-5.73677493311137E-16,1.09476442525376E-47,
1.));
#14534=DIRECTION('ref_axis',(-1.,4.74333763175827E-79,-5.73677493311137E-16));
#14535=DIRECTION('',(7.40148683083437E-16,0.,-1.));
#14536=DIRECTION('center_axis',(-5.73677493311137E-16,1.09476442525376E-47,
1.));
#14537=DIRECTION('ref_axis',(-1.,4.74333763175827E-79,-5.73677493311137E-16));
#14538=DIRECTION('center_axis',(-1.,0.,-7.40148683083437E-16));
#14539=DIRECTION('ref_axis',(0.,1.,0.));
#14540=DIRECTION('',(0.,1.,0.));
#14541=DIRECTION('',(7.40148683083437E-16,0.,-1.));
#14542=DIRECTION('',(0.,1.,0.));
#14543=DIRECTION('',(7.40148683083437E-16,0.,-1.));
#14544=DIRECTION('center_axis',(0.,1.,0.));
#14545=DIRECTION('ref_axis',(1.,0.,5.73677493311137E-16));
#14546=DIRECTION('',(1.,0.,5.73677493311137E-16));
#14547=DIRECTION('',(1.,0.,5.73677493311137E-16));
#14548=DIRECTION('',(7.40148683083437E-16,0.,-1.));
#14549=DIRECTION('center_axis',(1.,-3.55020428439413E-33,7.40148683083437E-16));
#14550=DIRECTION('ref_axis',(1.22343830028454E-32,-1.,-2.13262384275027E-17));
#14551=DIRECTION('',(1.22343830028454E-32,-1.,-2.13262384275027E-17));
#14552=DIRECTION('',(1.22343830028454E-32,-1.,-2.13262384275027E-17));
#14553=DIRECTION('',(7.40148683083437E-16,0.,-1.));
#14554=DIRECTION('center_axis',(0.,-1.,0.));
#14555=DIRECTION('ref_axis',(-1.,0.,-4.75766751584917E-16));
#14556=DIRECTION('',(-1.,0.,-4.75766751584917E-16));
#14557=DIRECTION('',(-1.,0.,-4.75766751584917E-16));
#14558=DIRECTION('center_axis',(-1.,0.,-7.40148683083437E-16));
#14559=DIRECTION('ref_axis',(0.,1.,0.));
#14560=DIRECTION('',(0.,1.,0.));
#14561=DIRECTION('',(7.40148683083437E-16,0.,-1.));
#14562=DIRECTION('',(0.,1.,0.));
#14563=DIRECTION('',(7.40148683083437E-16,0.,-1.));
#14564=DIRECTION('center_axis',(0.,1.,0.));
#14565=DIRECTION('ref_axis',(1.,0.,5.73677493311137E-16));
#14566=DIRECTION('',(1.,0.,5.73677493311137E-16));
#14567=DIRECTION('',(1.,0.,5.73677493311137E-16));
#14568=DIRECTION('',(7.40148683083437E-16,0.,-1.));
#14569=DIRECTION('center_axis',(1.,-3.55020428439413E-33,7.40148683083437E-16));
#14570=DIRECTION('ref_axis',(1.22343830028454E-32,-1.,-2.13262384275027E-17));
#14571=DIRECTION('',(1.22343830028454E-32,-1.,-2.13262384275027E-17));
#14572=DIRECTION('',(1.22343830028454E-32,-1.,-2.13262384275027E-17));
#14573=DIRECTION('',(7.40148683083437E-16,0.,-1.));
#14574=DIRECTION('center_axis',(0.,-1.,0.));
#14575=DIRECTION('ref_axis',(-1.,0.,-4.75766751584917E-16));
#14576=DIRECTION('',(-1.,0.,-4.75766751584917E-16));
#14577=DIRECTION('',(-1.,0.,-4.75766751584917E-16));
#14578=DIRECTION('center_axis',(7.40148683083437E-16,0.,-1.));
#14579=DIRECTION('ref_axis',(-1.,0.,-7.40148683083437E-16));
#14580=DIRECTION('center_axis',(-5.73677493311137E-16,1.09476442525376E-47,
1.));
#14581=DIRECTION('ref_axis',(-1.,4.74333763175827E-79,-5.73677493311137E-16));
#14582=DIRECTION('',(7.40148683083437E-16,0.,-1.));
#14583=DIRECTION('center_axis',(-5.73677493311137E-16,1.09476442525376E-47,
1.));
#14584=DIRECTION('ref_axis',(-1.,4.74333763175827E-79,-5.73677493311137E-16));
#14585=DIRECTION('center_axis',(7.40148683083437E-16,0.,-1.));
#14586=DIRECTION('ref_axis',(-1.,0.,-7.40148683083437E-16));
#14587=DIRECTION('center_axis',(-5.73677493311137E-16,1.09476442525376E-47,
1.));
#14588=DIRECTION('ref_axis',(-1.,4.74333763175827E-79,-5.73677493311137E-16));
#14589=DIRECTION('',(7.40148683083437E-16,0.,-1.));
#14590=DIRECTION('center_axis',(-5.73677493311137E-16,1.09476442525376E-47,
1.));
#14591=DIRECTION('ref_axis',(-1.,4.74333763175827E-79,-5.73677493311137E-16));
#14592=DIRECTION('center_axis',(-1.,0.,-7.40148683083437E-16));
#14593=DIRECTION('ref_axis',(0.,1.,0.));
#14594=DIRECTION('',(0.,1.,0.));
#14595=DIRECTION('',(7.40148683083437E-16,0.,-1.));
#14596=DIRECTION('',(0.,1.,0.));
#14597=DIRECTION('',(7.40148683083437E-16,0.,-1.));
#14598=DIRECTION('center_axis',(0.,1.,0.));
#14599=DIRECTION('ref_axis',(1.,0.,5.73677493311137E-16));
#14600=DIRECTION('',(1.,0.,5.73677493311137E-16));
#14601=DIRECTION('',(1.,0.,5.73677493311137E-16));
#14602=DIRECTION('',(7.40148683083437E-16,0.,-1.));
#14603=DIRECTION('center_axis',(1.,-3.55020428439413E-33,7.40148683083437E-16));
#14604=DIRECTION('ref_axis',(1.22343830028454E-32,-1.,-2.13262384275027E-17));
#14605=DIRECTION('',(1.22343830028454E-32,-1.,-2.13262384275027E-17));
#14606=DIRECTION('',(1.22343830028454E-32,-1.,-2.13262384275027E-17));
#14607=DIRECTION('',(7.40148683083437E-16,0.,-1.));
#14608=DIRECTION('center_axis',(0.,-1.,0.));
#14609=DIRECTION('ref_axis',(-1.,0.,-4.75766751584917E-16));
#14610=DIRECTION('',(-1.,0.,-4.75766751584917E-16));
#14611=DIRECTION('',(-1.,0.,-4.75766751584917E-16));
#14612=DIRECTION('center_axis',(7.40148683083437E-16,0.,-1.));
#14613=DIRECTION('ref_axis',(-1.,0.,-7.40148683083437E-16));
#14614=DIRECTION('center_axis',(-5.73677493311137E-16,1.09476442525376E-47,
1.));
#14615=DIRECTION('ref_axis',(-1.,4.74333763175827E-79,-5.73677493311137E-16));
#14616=DIRECTION('',(7.40148683083437E-16,0.,-1.));
#14617=DIRECTION('center_axis',(-5.73677493311137E-16,1.09476442525376E-47,
1.));
#14618=DIRECTION('ref_axis',(-1.,4.74333763175827E-79,-5.73677493311137E-16));
#14619=DIRECTION('center_axis',(7.40148683083437E-16,0.,-1.));
#14620=DIRECTION('ref_axis',(-1.,0.,-7.40148683083437E-16));
#14621=DIRECTION('center_axis',(-5.73677493311137E-16,1.09476442525376E-47,
1.));
#14622=DIRECTION('ref_axis',(-1.,4.74333763175827E-79,-5.73677493311137E-16));
#14623=DIRECTION('',(7.40148683083437E-16,0.,-1.));
#14624=DIRECTION('center_axis',(-5.73677493311137E-16,1.09476442525376E-47,
1.));
#14625=DIRECTION('ref_axis',(-1.,4.74333763175827E-79,-5.73677493311137E-16));
#14626=DIRECTION('center_axis',(0.,1.,0.));
#14627=DIRECTION('ref_axis',(1.,0.,5.73677493311137E-16));
#14628=DIRECTION('',(-1.,0.,-5.73677493311137E-16));
#14629=DIRECTION('',(7.40148683083437E-16,0.,-1.));
#14630=DIRECTION('',(1.,0.,5.73677493311137E-16));
#14631=DIRECTION('',(7.40148683083437E-16,0.,-1.));
#14632=DIRECTION('center_axis',(-1.,3.69640295643904E-34,-7.40148683083437E-16));
#14633=DIRECTION('ref_axis',(-1.27381992356653E-33,1.,2.22044604925031E-18));
#14634=DIRECTION('',(1.27381992356654E-33,-1.,-2.22044604925031E-18));
#14635=DIRECTION('',(-1.27381992356654E-33,1.,2.22044604925031E-18));
#14636=DIRECTION('',(7.40148683083437E-16,0.,-1.));
#14637=DIRECTION('center_axis',(0.,1.,0.));
#14638=DIRECTION('ref_axis',(1.,0.,3.77856009858697E-16));
#14639=DIRECTION('',(-1.,0.,-3.77856009858697E-16));
#14640=DIRECTION('',(1.,0.,3.77856009858697E-16));
#14641=DIRECTION('',(7.40148683083437E-16,0.,-1.));
#14642=DIRECTION('center_axis',(1.,2.22044604925031E-18,7.40148683083437E-16));
#14643=DIRECTION('ref_axis',(2.22044604925031E-18,-1.,1.27381992356654E-33));
#14644=DIRECTION('',(-2.22044604925031E-18,1.,-1.27381992356654E-33));
#14645=DIRECTION('',(2.22044604925031E-18,-1.,1.27381992356654E-33));
#14646=DIRECTION('',(7.40148683083437E-16,0.,-1.));
#14647=DIRECTION('center_axis',(0.,1.,0.));
#14648=DIRECTION('ref_axis',(1.,0.,5.73677493311137E-16));
#14649=DIRECTION('',(-1.,0.,-5.73677493311137E-16));
#14650=DIRECTION('',(1.,0.,5.73677493311137E-16));
#14651=DIRECTION('',(7.40148683083437E-16,0.,-1.));
#14652=DIRECTION('center_axis',(-1.,0.,-7.40148683083437E-16));
#14653=DIRECTION('ref_axis',(0.,1.,0.));
#14654=DIRECTION('',(0.,-1.,0.));
#14655=DIRECTION('',(0.,1.,0.));
#14656=DIRECTION('',(7.40148683083437E-16,0.,-1.));
#14657=DIRECTION('center_axis',(0.,1.,0.));
#14658=DIRECTION('ref_axis',(1.,0.,5.73677493311137E-16));
#14659=DIRECTION('',(-1.,0.,-5.73677493311137E-16));
#14660=DIRECTION('',(1.,0.,5.73677493311137E-16));
#14661=DIRECTION('',(7.40148683083437E-16,0.,-1.));
#14662=DIRECTION('center_axis',(1.,0.,7.40148683083437E-16));
#14663=DIRECTION('ref_axis',(0.,-1.,0.));
#14664=DIRECTION('',(0.,1.,0.));
#14665=DIRECTION('',(0.,-1.,0.));
#14666=DIRECTION('',(7.40148683083437E-16,0.,-1.));
#14667=DIRECTION('center_axis',(0.,1.,0.));
#14668=DIRECTION('ref_axis',(1.,0.,5.73677493311137E-16));
#14669=DIRECTION('',(-1.,0.,-5.73677493311137E-16));
#14670=DIRECTION('',(1.,0.,5.73677493311137E-16));
#14671=DIRECTION('',(7.40148683083437E-16,0.,-1.));
#14672=DIRECTION('center_axis',(7.40148683083437E-16,0.,-1.));
#14673=DIRECTION('ref_axis',(-1.,0.,-7.40148683083437E-16));
#14674=DIRECTION('center_axis',(5.73677493311137E-16,0.,-1.));
#14675=DIRECTION('ref_axis',(-1.,0.,-5.73677493311137E-16));
#14676=DIRECTION('center_axis',(5.73677493311137E-16,0.,-1.));
#14677=DIRECTION('ref_axis',(-1.,0.,-5.73677493311137E-16));
#14678=DIRECTION('',(7.40148683083437E-16,0.,-1.));
#14679=DIRECTION('center_axis',(-1.,0.,-7.40148683083437E-16));
#14680=DIRECTION('ref_axis',(0.,1.,0.));
#14681=DIRECTION('',(0.,-1.,0.));
#14682=DIRECTION('',(0.,1.,0.));
#14683=DIRECTION('',(7.40148683083437E-16,0.,-1.));
#14684=DIRECTION('center_axis',(7.40148683083437E-16,0.,-1.));
#14685=DIRECTION('ref_axis',(-8.88178419700122E-16,-1.,-6.57384087684173E-31));
#14686=DIRECTION('center_axis',(5.73677493311137E-16,0.,-1.));
#14687=DIRECTION('ref_axis',(-8.88178419700122E-16,-1.,-5.09527969426613E-31));
#14688=DIRECTION('center_axis',(5.73677493311137E-16,0.,-1.));
#14689=DIRECTION('ref_axis',(-8.88178419700122E-16,-1.,-5.09527969426613E-31));
#14690=DIRECTION('',(7.40148683083437E-16,0.,-1.));
#14691=DIRECTION('center_axis',(3.63363534449E-16,-1.,2.6894304150297E-31));
#14692=DIRECTION('ref_axis',(-1.,-3.63363534449E-16,-5.73677493311137E-16));
#14693=DIRECTION('',(1.,3.63363534449E-16,5.73677493311137E-16));
#14694=DIRECTION('',(-1.,-3.63363534449E-16,-5.73677493311137E-16));
#14695=DIRECTION('',(7.40148683083437E-16,0.,-1.));
#14696=DIRECTION('center_axis',(7.40148683083437E-16,0.,-1.));
#14697=DIRECTION('ref_axis',(1.,-1.77635683940025E-15,7.40148683083437E-16));
#14698=DIRECTION('center_axis',(5.73677493311137E-16,0.,-1.));
#14699=DIRECTION('ref_axis',(1.,-1.77635683940025E-15,5.73677493311137E-16));
#14700=DIRECTION('center_axis',(5.73677493311137E-16,0.,-1.));
#14701=DIRECTION('ref_axis',(1.,-1.77635683940025E-15,5.73677493311137E-16));
#14702=DIRECTION('',(7.40148683083437E-16,0.,-1.));
#14703=DIRECTION('center_axis',(1.,0.,7.40148683083437E-16));
#14704=DIRECTION('ref_axis',(0.,-1.,0.));
#14705=DIRECTION('',(0.,1.,0.));
#14706=DIRECTION('',(0.,-1.,0.));
#14707=DIRECTION('',(7.40148683083437E-16,0.,-1.));
#14708=DIRECTION('center_axis',(7.40148683083437E-16,0.,-1.));
#14709=DIRECTION('ref_axis',(-8.88178419700127E-16,1.,-6.57384087684177E-31));
#14710=DIRECTION('center_axis',(5.73677493311137E-16,0.,-1.));
#14711=DIRECTION('ref_axis',(-8.88178419700127E-16,1.,-5.09527969426616E-31));
#14712=DIRECTION('center_axis',(5.73677493311137E-16,0.,-1.));
#14713=DIRECTION('ref_axis',(-8.88178419700127E-16,1.,-5.09527969426616E-31));
#14714=DIRECTION('center_axis',(5.73677493311137E-16,0.,-1.));
#14715=DIRECTION('ref_axis',(-1.,0.,-5.73677493311137E-16));
#14716=DIRECTION('center_axis',(5.73677493311137E-16,0.,-1.));
#14717=DIRECTION('ref_axis',(-1.,0.,-5.73677493311137E-16));
#35480=CARTESIAN_POINT('',(0.,0.,0.));
#35481=CARTESIAN_POINT('Origin',(-25.5,-48.4435013582375,-10.));
#35482=CARTESIAN_POINT('',(-23.345,-48.4435013582375,-10.));
#35483=CARTESIAN_POINT('Origin',(-25.5,-48.4435013582375,-10.));
#35484=CARTESIAN_POINT('',(-23.345,-48.4435013582375,-13.));
#35485=CARTESIAN_POINT('',(-23.345,-48.4435013582375,-10.));
#35486=CARTESIAN_POINT('Origin',(-25.5,-48.4435013582375,-13.));
#35487=CARTESIAN_POINT('Origin',(-27.1652164893981,4.65750316817282,-10.));
#35488=CARTESIAN_POINT('',(-27.1652164893981,4.65750316817282,-10.));
#35489=CARTESIAN_POINT('',(-27.1652164893981,30.6870120381804,-10.));
#35490=CARTESIAN_POINT('',(-27.1652164893981,30.6870120381804,-10.));
#35491=CARTESIAN_POINT('',(-27.1652164893981,30.6870120381804,-13.));
#35492=CARTESIAN_POINT('',(-27.1652164893981,30.6870120381804,-10.));
#35493=CARTESIAN_POINT('',(-27.1652164893981,4.65750316817282,-13.));
#35494=CARTESIAN_POINT('',(-27.1652164893981,30.6870120381804,-13.));
#35495=CARTESIAN_POINT('',(-27.1652164893981,4.65750316817282,-10.));
#35496=CARTESIAN_POINT('Origin',(-32.8347835106019,4.65750316817282,-10.));
#35497=CARTESIAN_POINT('',(-32.8347835106019,4.65750316817282,-10.));
#35498=CARTESIAN_POINT('',(-27.1652164893981,4.65750316817282,-10.));
#35499=CARTESIAN_POINT('',(-32.8347835106019,4.65750316817282,-13.));
#35500=CARTESIAN_POINT('',(-27.1652164893981,4.65750316817282,-13.));
#35501=CARTESIAN_POINT('',(-32.8347835106019,4.65750316817282,-10.));
#35502=CARTESIAN_POINT('Origin',(-32.8347835106019,30.6870120381804,-10.));
#35503=CARTESIAN_POINT('',(-32.8347835106019,30.6870120381804,-10.));
#35504=CARTESIAN_POINT('',(-32.8347835106019,4.65750316817282,-10.));
#35505=CARTESIAN_POINT('',(-32.8347835106019,30.6870120381804,-13.));
#35506=CARTESIAN_POINT('',(-32.8347835106019,4.65750316817282,-13.));
#35507=CARTESIAN_POINT('',(-32.8347835106019,30.6870120381804,-10.));
#35508=CARTESIAN_POINT('Origin',(-27.1652164893981,30.6870120381804,-10.));
#35509=CARTESIAN_POINT('',(-32.8347835106019,30.6870120381804,-10.));
#35510=CARTESIAN_POINT('',(-32.8347835106019,30.6870120381804,-13.));
#35511=CARTESIAN_POINT('Origin',(2.83478351060189,4.65750316817282,-9.99999999999999));
#35512=CARTESIAN_POINT('',(2.83478351060189,4.65750316817282,-9.99999999999999));
#35513=CARTESIAN_POINT('',(2.83478351060189,30.6870120381804,-9.99999999999999));
#35514=CARTESIAN_POINT('',(2.83478351060189,30.6870120381804,-9.99999999999999));
#35515=CARTESIAN_POINT('',(2.83478351060189,30.6870120381804,-13.));
#35516=CARTESIAN_POINT('',(2.83478351060189,30.6870120381804,-9.99999999999999));
#35517=CARTESIAN_POINT('',(2.83478351060189,4.65750316817282,-13.));
#35518=CARTESIAN_POINT('',(2.8347835106019,30.6870120381804,-13.));
#35519=CARTESIAN_POINT('',(2.83478351060189,4.65750316817282,-9.99999999999999));
#35520=CARTESIAN_POINT('Origin',(-2.83478351060189,4.65750316817282,-9.99999999999999));
#35521=CARTESIAN_POINT('',(-2.83478351060189,4.65750316817282,-9.99999999999999));
#35522=CARTESIAN_POINT('',(2.83478351060189,4.65750316817282,-9.99999999999999));
#35523=CARTESIAN_POINT('',(-2.83478351060189,4.65750316817282,-13.));
#35524=CARTESIAN_POINT('',(2.8347835106019,4.65750316817282,-13.));
#35525=CARTESIAN_POINT('',(-2.83478351060189,4.65750316817282,-9.99999999999999));
#35526=CARTESIAN_POINT('Origin',(-2.83478351060189,30.6870120381804,-9.99999999999999));
#35527=CARTESIAN_POINT('',(-2.83478351060189,30.6870120381804,-9.99999999999999));
#35528=CARTESIAN_POINT('',(-2.83478351060189,4.65750316817282,-9.99999999999999));
#35529=CARTESIAN_POINT('',(-2.83478351060189,30.6870120381804,-13.));
#35530=CARTESIAN_POINT('',(-2.83478351060189,4.65750316817282,-13.));
#35531=CARTESIAN_POINT('',(-2.83478351060189,30.6870120381804,-9.99999999999999));
#35532=CARTESIAN_POINT('Origin',(2.83478351060189,30.6870120381804,-9.99999999999999));
#35533=CARTESIAN_POINT('',(-2.83478351060189,30.6870120381804,-9.99999999999999));
#35534=CARTESIAN_POINT('',(-2.83478351060189,30.6870120381804,-13.));
#35535=CARTESIAN_POINT('Origin',(5.50000000000001,-48.4435013582379,-9.99999999999999));
#35536=CARTESIAN_POINT('',(7.65500000000001,-48.4435013582379,-9.99999999999999));
#35537=CARTESIAN_POINT('Origin',(5.50000000000001,-48.4435013582379,-9.99999999999999));
#35538=CARTESIAN_POINT('',(7.65500000000001,-48.4435013582379,-13.));
#35539=CARTESIAN_POINT('',(7.65500000000001,-48.4435013582379,-9.99999999999999));
#35540=CARTESIAN_POINT('Origin',(5.50000000000001,-48.4435013582379,-13.));
#35541=CARTESIAN_POINT('Origin',(5.50000000000001,-17.4435013582379,-9.99999999999999));
#35542=CARTESIAN_POINT('',(7.65500000000001,-17.4435013582379,-9.99999999999999));
#35543=CARTESIAN_POINT('Origin',(5.50000000000001,-17.4435013582379,-9.99999999999999));
#35544=CARTESIAN_POINT('',(7.65500000000001,-17.4435013582379,-13.));
#35545=CARTESIAN_POINT('',(7.65500000000001,-17.4435013582379,-9.99999999999999));
#35546=CARTESIAN_POINT('Origin',(5.50000000000001,-17.4435013582379,-13.));
#35547=CARTESIAN_POINT('Origin',(-17.1652164893981,4.65750316817282,-10.));
#35548=CARTESIAN_POINT('',(-17.1652164893981,4.65750316817282,-10.));
#35549=CARTESIAN_POINT('',(-17.1652164893981,30.6870120381804,-10.));
#35550=CARTESIAN_POINT('',(-17.1652164893981,30.6870120381804,-10.));
#35551=CARTESIAN_POINT('',(-17.1652164893981,30.6870120381804,-13.));
#35552=CARTESIAN_POINT('',(-17.1652164893981,30.6870120381804,-10.));
#35553=CARTESIAN_POINT('',(-17.1652164893981,4.65750316817282,-13.));
#35554=CARTESIAN_POINT('',(-17.1652164893981,30.6870120381804,-13.));
#35555=CARTESIAN_POINT('',(-17.1652164893981,4.65750316817282,-10.));
#35556=CARTESIAN_POINT('Origin',(-22.8347835106019,4.65750316817282,-10.));
#35557=CARTESIAN_POINT('',(-22.8347835106019,4.65750316817282,-10.));
#35558=CARTESIAN_POINT('',(-17.1652164893981,4.65750316817282,-10.));
#35559=CARTESIAN_POINT('',(-22.8347835106019,4.65750316817282,-13.));
#35560=CARTESIAN_POINT('',(-17.1652164893981,4.65750316817282,-13.));
#35561=CARTESIAN_POINT('',(-22.8347835106019,4.65750316817282,-10.));
#35562=CARTESIAN_POINT('Origin',(-22.8347835106019,30.6870120381804,-10.));
#35563=CARTESIAN_POINT('',(-22.8347835106019,30.6870120381804,-10.));
#35564=CARTESIAN_POINT('',(-22.8347835106019,4.65750316817282,-10.));
#35565=CARTESIAN_POINT('',(-22.8347835106019,30.6870120381804,-13.));
#35566=CARTESIAN_POINT('',(-22.8347835106019,4.65750316817282,-13.));
#35567=CARTESIAN_POINT('',(-22.8347835106019,30.6870120381804,-10.));
#35568=CARTESIAN_POINT('Origin',(-17.1652164893981,30.6870120381804,-10.));
#35569=CARTESIAN_POINT('',(-22.8347835106019,30.6870120381804,-10.));
#35570=CARTESIAN_POINT('',(-22.8347835106019,30.6870120381804,-13.));
#35571=CARTESIAN_POINT('Origin',(-10.,-32.9435013582377,-10.));
#35572=CARTESIAN_POINT('',(1.493,-32.9435013582377,-9.99999999999999));
#35573=CARTESIAN_POINT('Origin',(-10.,-32.9435013582377,-10.));
#35574=CARTESIAN_POINT('',(1.493,-32.9435013582377,-13.));
#35575=CARTESIAN_POINT('',(1.493,-32.9435013582377,-9.99999999999999));
#35576=CARTESIAN_POINT('Origin',(-9.99999999999999,-32.9435013582377,-13.));
#35577=CARTESIAN_POINT('Origin',(-25.5,-17.4435013582375,-10.));
#35578=CARTESIAN_POINT('',(-23.345,-17.4435013582375,-10.));
#35579=CARTESIAN_POINT('Origin',(-25.5,-17.4435013582375,-10.));
#35580=CARTESIAN_POINT('',(-23.345,-17.4435013582375,-13.));
#35581=CARTESIAN_POINT('',(-23.345,-17.4435013582375,-10.));
#35582=CARTESIAN_POINT('Origin',(-25.5,-17.4435013582375,-13.));
#35583=CARTESIAN_POINT('Origin',(12.8347835106019,35.2970569134824,-9.99999999999998));
#35584=CARTESIAN_POINT('',(15.,35.2970569134824,-9.99999999999998));
#35585=CARTESIAN_POINT('',(12.8347835106019,35.2970569134824,-9.99999999999998));
#35586=CARTESIAN_POINT('',(15.,35.2970569134824,-9.99999999999998));
#35587=CARTESIAN_POINT('',(15.,35.2970569134824,-13.));
#35588=CARTESIAN_POINT('',(15.,35.2970569134824,-9.99999999999998));
#35589=CARTESIAN_POINT('',(12.8347835106019,35.2970569134824,-13.));
#35590=CARTESIAN_POINT('',(15.,35.2970569134824,-13.));
#35591=CARTESIAN_POINT('',(12.8347835106019,35.2970569134824,-9.99999999999998));
#35592=CARTESIAN_POINT('Origin',(12.8347835106019,0.,-9.99999999999998));
#35593=CARTESIAN_POINT('',(12.8347835106019,0.,-9.99999999999998));
#35594=CARTESIAN_POINT('',(12.8347835106019,500.,-9.99999999999998));
#35595=CARTESIAN_POINT('',(12.8347835106019,0.,-13.));
#35596=CARTESIAN_POINT('',(12.8347835106019,500.,-13.));
#35597=CARTESIAN_POINT('',(12.8347835106019,0.,-9.99999999999998));
#35598=CARTESIAN_POINT('Origin',(7.16521648939811,0.,-9.99999999999999));
#35599=CARTESIAN_POINT('',(7.16521648939811,0.,-9.99999999999999));
#35600=CARTESIAN_POINT('',(12.8347835106019,0.,-9.99999999999998));
#35601=CARTESIAN_POINT('',(7.16521648939812,0.,-13.));
#35602=CARTESIAN_POINT('',(12.8347835106019,0.,-13.));
#35603=CARTESIAN_POINT('',(7.16521648939811,0.,-9.99999999999999));
#35604=CARTESIAN_POINT('Origin',(7.16521648939811,35.2970569134824,-9.99999999999999));
#35605=CARTESIAN_POINT('',(7.16521648939811,35.2970569134824,-9.99999999999999));
#35606=CARTESIAN_POINT('',(7.16521648939811,0.,-9.99999999999999));
#35607=CARTESIAN_POINT('',(7.16521648939812,35.2970569134824,-13.));
#35608=CARTESIAN_POINT('',(7.16521648939812,0.,-13.));
#35609=CARTESIAN_POINT('',(7.16521648939811,35.2970569134824,-9.99999999999999));
#35610=CARTESIAN_POINT('Origin',(-7.16521648939811,35.2970569134824,-10.));
#35611=CARTESIAN_POINT('',(-7.16521648939811,35.2970569134824,-10.));
#35612=CARTESIAN_POINT('',(15.,35.2970569134824,-9.99999999999998));
#35613=CARTESIAN_POINT('',(-7.16521648939811,35.2970569134824,-13.));
#35614=CARTESIAN_POINT('',(15.,35.2970569134824,-13.));
#35615=CARTESIAN_POINT('',(-7.16521648939811,35.2970569134824,-10.));
#35616=CARTESIAN_POINT('Origin',(-7.16521648939811,0.,-10.));
#35617=CARTESIAN_POINT('',(-7.16521648939811,0.,-10.));
#35618=CARTESIAN_POINT('',(-7.16521648939811,500.,-10.));
#35619=CARTESIAN_POINT('',(-7.16521648939811,0.,-13.));
#35620=CARTESIAN_POINT('',(-7.1652164893981,500.,-13.));
#35621=CARTESIAN_POINT('',(-7.16521648939811,0.,-10.));
#35622=CARTESIAN_POINT('Origin',(-12.8347835106019,0.,-10.));
#35623=CARTESIAN_POINT('',(-12.8347835106019,0.,-10.));
#35624=CARTESIAN_POINT('',(-7.16521648939811,0.,-10.));
#35625=CARTESIAN_POINT('',(-12.8347835106019,0.,-13.));
#35626=CARTESIAN_POINT('',(-7.1652164893981,0.,-13.));
#35627=CARTESIAN_POINT('',(-12.8347835106019,0.,-10.));
#35628=CARTESIAN_POINT('Origin',(-12.8347835106019,35.2970569134824,-10.));
#35629=CARTESIAN_POINT('',(-12.8347835106019,35.2970569134824,-10.));
#35630=CARTESIAN_POINT('',(-12.8347835106019,0.,-10.));
#35631=CARTESIAN_POINT('',(-12.8347835106019,35.2970569134824,-13.));
#35632=CARTESIAN_POINT('',(-12.8347835106019,0.,-13.));
#35633=CARTESIAN_POINT('',(-12.8347835106019,35.2970569134824,-10.));
#35634=CARTESIAN_POINT('Origin',(-33.8864916534318,35.2970569134824,-10.));
#35635=CARTESIAN_POINT('',(-33.8864916534318,35.2970569134824,-10.));
#35636=CARTESIAN_POINT('',(15.,35.2970569134824,-9.99999999999998));
#35637=CARTESIAN_POINT('',(-33.8864916534318,35.2970569134824,-13.));
#35638=CARTESIAN_POINT('',(15.,35.2970569134824,-13.));
#35639=CARTESIAN_POINT('',(-33.8864916534318,35.2970569134824,-10.));
#35640=CARTESIAN_POINT('Origin',(-33.8864916534318,30.2970569134824,-10.));
#35641=CARTESIAN_POINT('',(-38.8864916534318,30.2970569134824,-10.));
#35642=CARTESIAN_POINT('Origin',(-33.8864916534318,30.2970569134824,-10.));
#35643=CARTESIAN_POINT('',(-38.8864916534318,30.2970569134824,-13.));
#35644=CARTESIAN_POINT('Origin',(-33.8864916534318,30.2970569134824,-13.));
#35645=CARTESIAN_POINT('',(-38.8864916534318,30.2970569134824,-10.));
#35646=CARTESIAN_POINT('Origin',(-38.8864916534318,-56.2946587134524,-10.));
#35647=CARTESIAN_POINT('',(-38.8864916534318,-56.2946587134524,-10.));
#35648=CARTESIAN_POINT('',(-38.8864916534318,30.2970569134824,-10.));
#35649=CARTESIAN_POINT('',(-38.8864916534318,-56.2946587134524,-13.));
#35650=CARTESIAN_POINT('',(-38.8864916534318,30.2970569134824,-13.));
#35651=CARTESIAN_POINT('',(-38.8864916534318,-56.2946587134524,-10.));
#35652=CARTESIAN_POINT('Origin',(-33.8864916534318,-56.2946587134524,-10.));
#35653=CARTESIAN_POINT('',(-33.8864916534318,-61.2946587134525,-10.));
#35654=CARTESIAN_POINT('Origin',(-33.8864916534318,-56.2946587134524,-10.));
#35655=CARTESIAN_POINT('',(-33.8864916534318,-61.2946587134525,-13.));
#35656=CARTESIAN_POINT('Origin',(-33.8864916534318,-56.2946587134524,-13.));
#35657=CARTESIAN_POINT('',(-33.8864916534318,-61.2946587134525,-10.));
#35658=CARTESIAN_POINT('Origin',(15.,-61.2946587134524,-9.99999999999998));
#35659=CARTESIAN_POINT('',(15.,-61.2946587134524,-9.99999999999998));
#35660=CARTESIAN_POINT('',(-33.8864916534318,-61.2946587134525,-10.));
#35661=CARTESIAN_POINT('',(15.,-61.2946587134524,-13.));
#35662=CARTESIAN_POINT('',(-33.8864916534318,-61.2946587134525,-13.));
#35663=CARTESIAN_POINT('',(15.,-61.2946587134524,-9.99999999999998));
#35664=CARTESIAN_POINT('Origin',(15.,-56.2946587134524,-9.99999999999998));
#35665=CARTESIAN_POINT('',(20.,-56.2946587134525,-9.99999999999998));
#35666=CARTESIAN_POINT('Origin',(15.,-56.2946587134524,-9.99999999999998));
#35667=CARTESIAN_POINT('',(20.,-56.2946587134525,-13.));
#35668=CARTESIAN_POINT('Origin',(15.,-56.2946587134524,-13.));
#35669=CARTESIAN_POINT('',(20.,-56.2946587134525,-9.99999999999998));
#35670=CARTESIAN_POINT('Origin',(20.,30.2970569134825,-9.99999999999998));
#35671=CARTESIAN_POINT('',(20.,30.2970569134825,-9.99999999999998));
#35672=CARTESIAN_POINT('',(20.,-56.2946587134525,-9.99999999999998));
#35673=CARTESIAN_POINT('',(20.,30.2970569134825,-13.));
#35674=CARTESIAN_POINT('',(20.,-56.2946587134525,-13.));
#35675=CARTESIAN_POINT('',(20.,30.2970569134825,-9.99999999999998));
#35676=CARTESIAN_POINT('Origin',(15.,30.2970569134825,-9.99999999999998));
#35677=CARTESIAN_POINT('Origin',(15.,30.2970569134825,-9.99999999999998));
#35678=CARTESIAN_POINT('Origin',(15.,30.2970569134825,-13.));
#35679=CARTESIAN_POINT('Origin',(-9.44324582671591,-12.998800899985,-13.));
#35680=CARTESIAN_POINT('Origin',(-9.44324582671591,-12.998800899985,-10.));
#36438=UNCERTAINTY_MEASURE_WITH_UNIT(LENGTH_MEASURE(0.01),#36461,
'DISTANCE_ACCURACY_VALUE',
'Maximum model space distance between geometric entities at asserted c
onnectivities');
#36444=UNCERTAINTY_MEASURE_WITH_UNIT(LENGTH_MEASURE(0.01),#36461,
'DISTANCE_ACCURACY_VALUE',
'Maximum model space distance between geometric entities at asserted c
onnectivities');
#36454=(
GEOMETRIC_REPRESENTATION_CONTEXT(3)
GLOBAL_UNCERTAINTY_ASSIGNED_CONTEXT((#36438))
GLOBAL_UNIT_ASSIGNED_CONTEXT((#36461,#36463,#36464))
REPRESENTATION_CONTEXT('','3D')
);
#36460=(
GEOMETRIC_REPRESENTATION_CONTEXT(3)
GLOBAL_UNCERTAINTY_ASSIGNED_CONTEXT((#36444))
GLOBAL_UNIT_ASSIGNED_CONTEXT((#36461,#36463,#36464))
REPRESENTATION_CONTEXT('','3D')
);
#36461=(
LENGTH_UNIT()
NAMED_UNIT(*)
SI_UNIT(.MILLI.,.METRE.)
);
#36463=(
NAMED_UNIT(*)
PLANE_ANGLE_UNIT()
SI_UNIT($,.RADIAN.)
);
#36464=(
NAMED_UNIT(*)
SI_UNIT($,.STERADIAN.)
SOLID_ANGLE_UNIT()
);
#36474=SHAPE_DEFINITION_REPRESENTATION(#36494,#36525);
#36494=PRODUCT_DEFINITION_SHAPE('',$,#36541);
#36525=SHAPE_REPRESENTATION('',(#12135),#36454);
#36531=PRODUCT_DEFINITION_CONTEXT('part definition',#36578,'design');
#36541=PRODUCT_DEFINITION('Bracket_Motor','Bracket_Motor',#36556,#36531);
#36556=PRODUCT_DEFINITION_FORMATION('',$,#36589);
#36578=APPLICATION_CONTEXT(
'Core Data for Automotive Mechanical Design Process');
#36579=PRODUCT_CONTEXT('part definition',#36578,'mechanical');
#36589=PRODUCT('Bracket_Motor','Bracket_Motor',$,(#36579));
#36596=PRESENTATION_STYLE_ASSIGNMENT((#36601));
#36601=SURFACE_STYLE_USAGE(.BOTH.,#36606);
#36606=SURFACE_SIDE_STYLE('',(#36611));
#36611=SURFACE_STYLE_FILL_AREA(#36616);
#36616=FILL_AREA_STYLE('Opaque(160,160,160)',(#36621));
#36621=FILL_AREA_STYLE_COLOUR('Opaque(160,160,160)',#36626);
#36626=COLOUR_RGB('Opaque(160,160,160)', 0.09019608, 0.27058824, 0.51372549);
ENDSEC;
END-ISO-10303-21;
